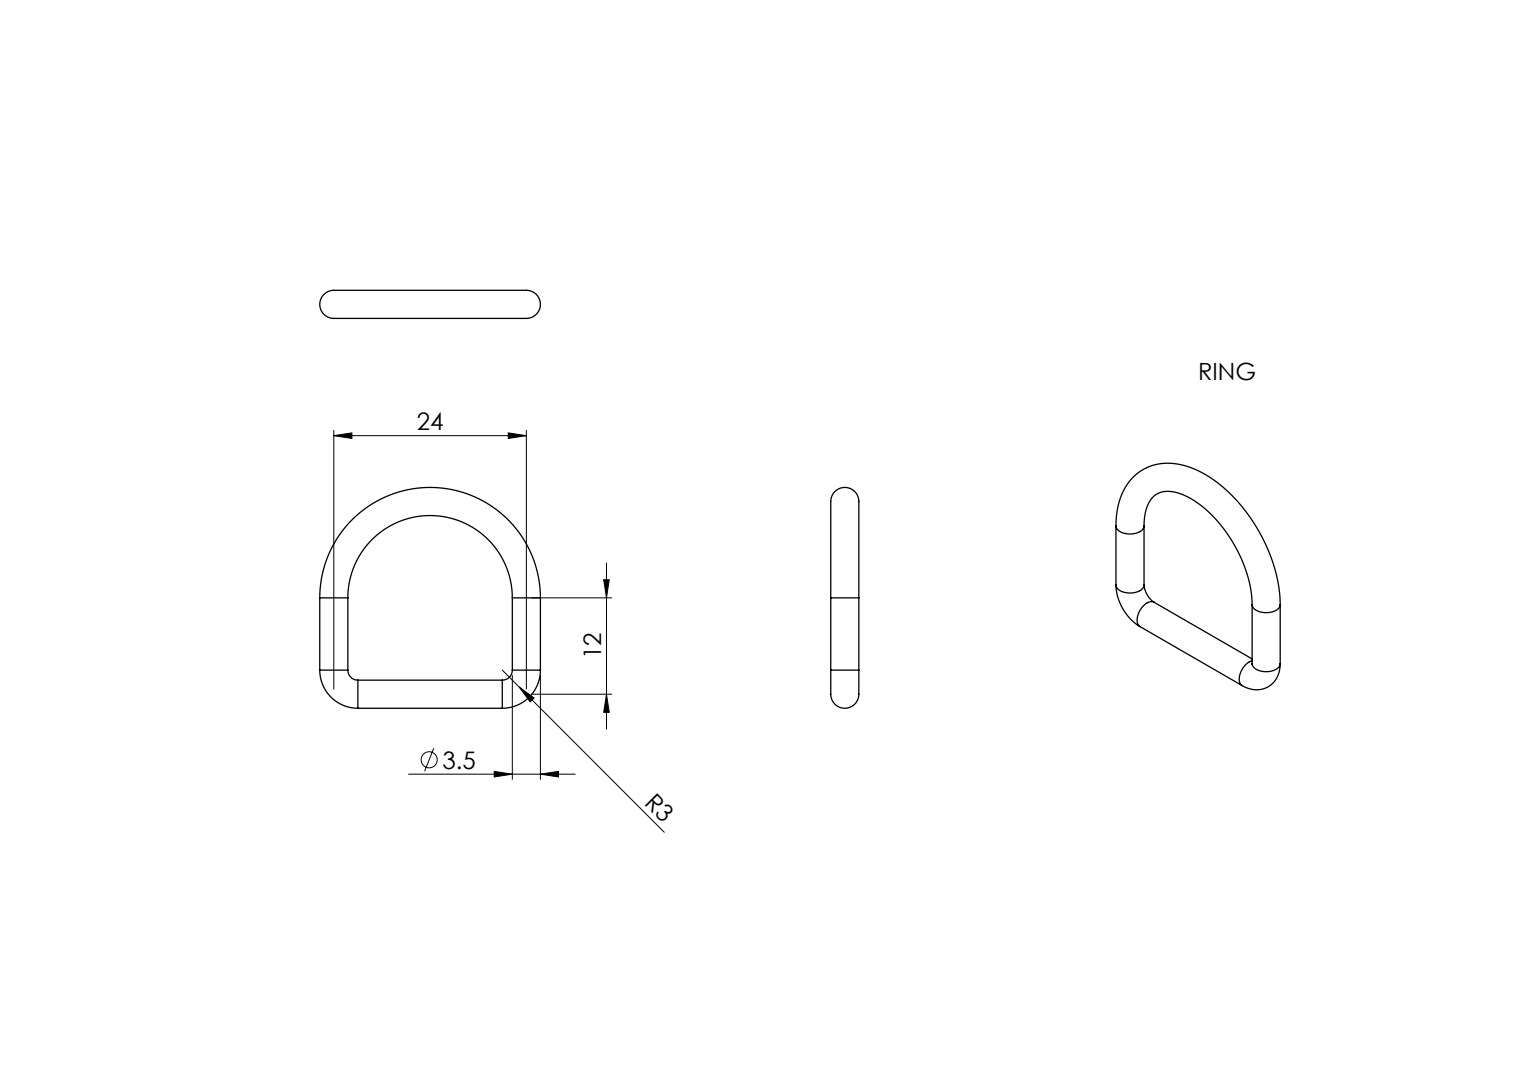
ISO-10303-21;
HEADER;
FILE_DESCRIPTION (('STEP AP214'),
    '1' );
FILE_NAME ('ring.step',
    '2026-10-26T11:20:31',
    ( '' ),
    ( '' ),
    'SwSTEP 2.0',
    'SolidWorks 2026',
    '' );
FILE_SCHEMA (( 'AUTOMOTIVE_DESIGN' ));
ENDSEC;

DATA;
#29=VERTEX_POINT ( 'NONE', #4130 ) ;
#30=CARTESIAN_POINT ( 'NONE',  ( -8.999999999999998224, 36.00000000000000711, 0.000000000000000000 ) ) ;
#48=CIRCLE ( 'NONE', #1190, 1.749999999999999778 ) ;
#49=DIRECTION ( 'NONE',  ( -0.000000000000000000, -0.000000000000000000, -1.000000000000000000 ) ) ;
#66=TOROIDAL_SURFACE ( 'NONE', #1579, 12.00000000000000000, 1.749999999999999778 ) ;
#77=CIRCLE ( 'NONE', #3336, 1.749999999999999778 ) ;
#79=UNCERTAINTY_MEASURE_WITH_UNIT (LENGTH_MEASURE( 1.000000000000000082E-05 ), #706, 'distance_accuracy_value', 'NONE');
#80=DIRECTION ( 'NONE',  ( 1.000000000000000000, -1.621111868633889227E-15, 0.000000000000000000 ) ) ;
#88=FACE_OUTER_BOUND ( 'NONE', #3234, .T. ) ;
#100=CIRCLE ( 'NONE', #1688, 1.749999999999999778 ) ;
#121=( NAMED_UNIT ( * ) PLANE_ANGLE_UNIT ( ) SI_UNIT ( $, .RADIAN. ) );
#148=ORIENTED_EDGE ( 'NONE', *, *, #3909, .T. ) ;
#150=ORIENTED_EDGE ( 'NONE', *, *, #4580, .T. ) ;
#175=CARTESIAN_POINT ( 'NONE',  ( -1.734723475976807094E-15, 45.00000000000000000, 0.000000000000000000 ) ) ;
#218=CIRCLE ( 'NONE', #2726, 1.250000000000002887 ) ;
#228=ORIENTED_EDGE ( 'NONE', *, *, #457, .T. ) ;
#244=CARTESIAN_POINT ( 'NONE',  ( 8.999999999999996447, 34.74999999999999289, 2.143131898507865832E-16 ) ) ;
#261=DIRECTION ( 'NONE',  ( 0.000000000000000000, 0.000000000000000000, 1.000000000000000000 ) ) ;
#303=CARTESIAN_POINT ( 'NONE',  ( 9.000000000000003553, 36.00000000000000000, 2.143131898507868051E-16 ) ) ;
#327=ORIENTED_EDGE ( 'NONE', *, *, #457, .F. ) ;
#344=SHAPE_DEFINITION_REPRESENTATION ( #546, #4641 ) ;
#347=DIRECTION ( 'NONE',  ( -1.000000000000000000, -0.000000000000000000, -0.000000000000000000 ) ) ;
#357=DIRECTION ( 'NONE',  ( -0.000000000000000000, -0.000000000000000000, -1.000000000000000000 ) ) ;
#372=EDGE_LOOP ( 'NONE', ( #1130, #2275, #3372, #4073 ) ) ;
#376=ORIENTED_EDGE ( 'NONE', *, *, #4634, .F. ) ;
#379=LINE ( 'NONE', #4051, #4102 ) ;
#430=DIRECTION ( 'NONE',  ( -1.000000000000000000, 0.000000000000000000, 0.000000000000000000 ) ) ;
#455=CARTESIAN_POINT ( 'NONE',  ( 8.999999999999980460, 32.99999999999999289, 0.000000000000000000 ) ) ;
#457=EDGE_CURVE ( 'NONE', #2385, #2339, #3083, .T. ) ;
#459=EDGE_CURVE ( 'NONE', #2022, #1315, #48, .T. ) ;
#469=EDGE_CURVE ( 'NONE', #29, #4376, #2892, .T. ) ;
#481=UNCERTAINTY_MEASURE_WITH_UNIT (LENGTH_MEASURE( 1.000000000000000082E-05 ), #3442, 'distance_accuracy_value', 'NONE');
#489=CIRCLE ( 'NONE', #2768, 1.750000000000001554 ) ;
#493=CYLINDRICAL_SURFACE ( 'NONE', #995, 1.749999999999999778 ) ;
#522=FILL_AREA_STYLE_COLOUR ( '', #3240 ) ;
#529=( GEOMETRIC_REPRESENTATION_CONTEXT ( 3 ) GLOBAL_UNCERTAINTY_ASSIGNED_CONTEXT ( ( #79 ) ) GLOBAL_UNIT_ASSIGNED_CONTEXT ( ( #706, #2210, #4340 ) ) REPRESENTATION_CONTEXT ( 'NONE', 'WORKASPACE' ) );
#532=CIRCLE ( 'NONE', #3102, 1.750000000000001554 ) ;
#545=CARTESIAN_POINT ( 'NONE',  ( -8.999999999999998224, 36.00000000000000711, 2.143131898507868051E-16 ) ) ;
#546=PRODUCT_DEFINITION_SHAPE ( 'NONE', 'NONE',  #1816 ) ;
#548=EDGE_LOOP ( 'NONE', ( #758, #4521, #1673, #3066 ) ) ;
#579=EDGE_CURVE ( 'NONE', #3730, #2339, #1566, .T. ) ;
#614=VERTEX_POINT ( 'NONE', #1484 ) ;
#615=DIRECTION ( 'NONE',  ( 8.921435019309286191E-15, 1.000000000000000000, 0.000000000000000000 ) ) ;
#619=DIRECTION ( 'NONE',  ( 1.000000000000000000, 0.000000000000000000, 0.000000000000000000 ) ) ;
#636=EDGE_LOOP ( 'NONE', ( #2161, #3608, #3305, #4453 ) ) ;
#655=CARTESIAN_POINT ( 'NONE',  ( 12.00000000000000178, 36.00000000000000000, 0.000000000000000000 ) ) ;
#660=SURFACE_SIDE_STYLE ('',( #3422 ) ) ;
#684=PRODUCT_CONTEXT ( 'NONE', #3739, 'mechanical' ) ;
#690=CARTESIAN_POINT ( 'NONE',  ( 8.999999999999980460, 32.99999999999999289, -1.749999999999999778 ) ) ;
#700=EDGE_LOOP ( 'NONE', ( #4101, #4550, #228, #2693, #3793 ) ) ;
#702=CARTESIAN_POINT ( 'NONE',  ( 9.000000000000003553, 36.00000000000000000, 0.000000000000000000 ) ) ;
#706=( LENGTH_UNIT ( ) NAMED_UNIT ( * ) SI_UNIT ( .MILLI., .METRE. ) );
#713=CARTESIAN_POINT ( 'NONE',  ( 10.25000000000001954, 44.99999999999999289, 2.143131898507868051E-16 ) ) ;
#733=DIRECTION ( 'NONE',  ( 5.782411586589374402E-16, -1.000000000000000000, 0.000000000000000000 ) ) ;
#744=DIRECTION ( 'NONE',  ( -0.000000000000000000, -0.000000000000000000, -1.000000000000000000 ) ) ;
#758=ORIENTED_EDGE ( 'NONE', *, *, #1941, .F. ) ;
#762=DIRECTION ( 'NONE',  ( 1.000000000000000000, -8.560005772541128451E-15, 0.000000000000000000 ) ) ;
#767=CARTESIAN_POINT ( 'NONE',  ( -1.734723475976807094E-15, 45.00000000000000000, 2.143131898507868051E-16 ) ) ;
#768=AXIS2_PLACEMENT_3D ( 'NONE', #3232, #762, #3279 ) ;
#780=CARTESIAN_POINT ( 'NONE',  ( -13.75000000000000178, 36.00000000000001421, 0.000000000000000000 ) ) ;
#787=EDGE_LOOP ( 'NONE', ( #3435, #2481, #1946, #2209, #849 ) ) ;
#836=ORIENTED_EDGE ( 'NONE', *, *, #2413, .T. ) ;
#838=DIRECTION ( 'NONE',  ( 1.000000000000000000, 0.000000000000000000, 0.000000000000000000 ) ) ;
#849=ORIENTED_EDGE ( 'NONE', *, *, #1941, .T. ) ;
#853=AXIS2_PLACEMENT_3D ( 'NONE', #455, #2640, #4104 ) ;
#859=DIRECTION ( 'NONE',  ( -1.428364815747576977E-15, -1.000000000000000000, 0.000000000000000000 ) ) ;
#918=CYLINDRICAL_SURFACE ( 'NONE', #4520, 1.749999999999999778 ) ;
#927=DIRECTION ( 'NONE',  ( 1.621111868633889227E-15, 1.000000000000000000, 0.000000000000000000 ) ) ;
#929=PRESENTATION_STYLE_ASSIGNMENT (( #2652 ) ) ;
#945=DIRECTION ( 'NONE',  ( 1.000000000000000000, 0.000000000000000000, 0.000000000000000000 ) ) ;
#955=AXIS2_PLACEMENT_3D ( 'NONE', #1133, #2645, #3717 ) ;
#958=ORIENTED_EDGE ( 'NONE', *, *, #4634, .T. ) ;
#962=AXIS2_PLACEMENT_3D ( 'NONE', #3454, #3122, #3098 ) ;
#966=CARTESIAN_POINT ( 'NONE',  ( -8.999999999999969802, 34.74999999999999289, 2.143131898507857451E-16 ) ) ;
#971=VECTOR ( 'NONE', #2847, 1000.000000000000000 ) ;
#976=FACE_OUTER_BOUND ( 'NONE', #2756, .T. ) ;
#982=CIRCLE ( 'NONE', #4392, 1.749999999999999778 ) ;
#995=AXIS2_PLACEMENT_3D ( 'NONE', #2650, #4193, #2333 ) ;
#1008=DIRECTION ( 'NONE',  ( 1.000000000000000000, 0.000000000000000000, 0.000000000000000000 ) ) ;
#1032=CARTESIAN_POINT ( 'NONE',  ( 13.75000000000000178, 36.00000000000000000, 0.000000000000000000 ) ) ;
#1057=AXIS2_PLACEMENT_3D ( 'NONE', #767, #357, #430 ) ;
#1058=DIRECTION ( 'NONE',  ( 1.621111868633889227E-15, 1.000000000000000000, 0.000000000000000000 ) ) ;
#1070=EDGE_CURVE ( 'NONE', #4401, #3730, #2816, .T. ) ;
#1083=CLOSED_SHELL ( 'NONE', ( #1845, #4127, #2356, #3065, #4322, #2721, #4192, #3598, #1324, #1603, #2660, #3233 ) ) ;
#1087=DIRECTION ( 'NONE',  ( -1.000000000000000000, 0.000000000000000000, 0.000000000000000000 ) ) ;
#1116=PRODUCT_DEFINITION_FORMATION_WITH_SPECIFIED_SOURCE ( 'ANY', '', #2031, .NOT_KNOWN. ) ;
#1130=ORIENTED_EDGE ( 'NONE', *, *, #4580, .F. ) ;
#1133=CARTESIAN_POINT ( 'NONE',  ( -8.999999999999998224, 36.00000000000000711, 0.000000000000000000 ) ) ;
#1144=( NAMED_UNIT ( * ) PLANE_ANGLE_UNIT ( ) SI_UNIT ( $, .RADIAN. ) );
#1150=TOROIDAL_SURFACE ( 'NONE', #1749, 3.000000000000002665, 1.749999999999999778 ) ;
#1171=CARTESIAN_POINT ( 'NONE',  ( -12.00000000000000178, 36.00000000000001421, 0.000000000000000000 ) ) ;
#1177=EDGE_CURVE ( 'NONE', #3258, #4401, #3344, .T. ) ;
#1178=AXIS2_PLACEMENT_3D ( 'NONE', #175, #3762, #2028 ) ;
#1190=AXIS2_PLACEMENT_3D ( 'NONE', #2109, #1819, #1396 ) ;
#1202=AXIS2_PLACEMENT_3D ( 'NONE', #4076, #80, #3046 ) ;
#1208=AXIS2_PLACEMENT_3D ( 'NONE', #1938, #1277, #945 ) ;
#1237=( NAMED_UNIT ( * ) SI_UNIT ( $, .STERADIAN. ) SOLID_ANGLE_UNIT ( ) );
#1252=CARTESIAN_POINT ( 'NONE',  ( -13.75000000000000178, 44.99999999999999289, 0.000000000000000000 ) ) ;
#1277=DIRECTION ( 'NONE',  ( 5.782411586589374402E-16, -1.000000000000000000, 0.000000000000000000 ) ) ;
#1286=CARTESIAN_POINT ( 'NONE',  ( 12.00000000000000178, 36.00000000000000000, 0.000000000000000000 ) ) ;
#1296=DIRECTION ( 'NONE',  ( -0.000000000000000000, -0.000000000000000000, -1.000000000000000000 ) ) ;
#1298=AXIS2_PLACEMENT_3D ( 'NONE', #3596, #3193, #1008 ) ;
#1313=ORIENTED_EDGE ( 'NONE', *, *, #3981, .T. ) ;
#1315=VERTEX_POINT ( 'NONE', #3475 ) ;
#1324=ADVANCED_FACE ( 'NONE', ( #3097 ), #1150, .T. ) ;
#1347=DIRECTION ( 'NONE',  ( 1.982541115402063335E-15, 1.000000000000000000, 0.000000000000000000 ) ) ;
#1365=FACE_OUTER_BOUND ( 'NONE', #1708, .T. ) ;
#1396=DIRECTION ( 'NONE',  ( -1.000000000000000000, 0.000000000000000000, 0.000000000000000000 ) ) ;
#1401=AXIS2_PLACEMENT_3D ( 'NONE', #655, #1058, #3239 ) ;
#1431=DIRECTION ( 'NONE',  ( 1.000000000000000000, 0.000000000000000000, 0.000000000000000000 ) ) ;
#1472=TOROIDAL_SURFACE ( 'NONE', #955, 3.000000000000002665, 1.749999999999999778 ) ;
#1484=CARTESIAN_POINT ( 'NONE',  ( -8.999999999999973355, 32.99999999999999289, 1.749999999999999778 ) ) ;
#1511=( NAMED_UNIT ( * ) SI_UNIT ( $, .STERADIAN. ) SOLID_ANGLE_UNIT ( ) );
#1536=ORIENTED_EDGE ( 'NONE', *, *, #3804, .T. ) ;
#1554=AXIS2_PLACEMENT_3D ( 'NONE', #3843, #2742, #3798 ) ;
#1566=CIRCLE ( 'NONE', #3162, 1.750000000000001554 ) ;
#1579=AXIS2_PLACEMENT_3D ( 'NONE', #1616, #2659, #4176 ) ;
#1603=ADVANCED_FACE ( 'NONE', ( #3825 ), #493, .T. ) ;
#1609=AXIS2_PLACEMENT_3D ( 'NONE', #702, #744, #2587 ) ;
#1616=CARTESIAN_POINT ( 'NONE',  ( -1.734723475976807094E-15, 45.00000000000000000, 0.000000000000000000 ) ) ;
#1628=LINE ( 'NONE', #4189, #3221 ) ;
#1632=SHAPE_REPRESENTATION_RELATIONSHIP ( 'NONE' , 'NONE' ,  #4641, #4382 ) ;
#1643=VERTEX_POINT ( 'NONE', #3398 ) ;
#1663=DIRECTION ( 'NONE',  ( -1.000000000000000000, -0.000000000000000000, -0.000000000000000000 ) ) ;
#1664=CARTESIAN_POINT ( 'NONE',  ( -8.999999999999998224, 36.00000000000000711, 0.000000000000000000 ) ) ;
#1673=ORIENTED_EDGE ( 'NONE', *, *, #3531, .T. ) ;
#1685=ORIENTED_EDGE ( 'NONE', *, *, #3593, .T. ) ;
#1688=AXIS2_PLACEMENT_3D ( 'NONE', #4667, #1726, #4615 ) ;
#1703=EDGE_CURVE ( 'NONE', #1315, #2022, #100, .T. ) ;
#1708=EDGE_LOOP ( 'NONE', ( #3770, #2507, #1313, #2365 ) ) ;
#1712=DIRECTION ( 'NONE',  ( 0.000000000000000000, 0.000000000000000000, 1.000000000000000000 ) ) ;
#1717=CARTESIAN_POINT ( 'NONE',  ( 8.999999999999966249, 31.24999999999999645, 0.000000000000000000 ) ) ;
#1726=DIRECTION ( 'NONE',  ( 1.621111868633889227E-15, 1.000000000000000000, 0.000000000000000000 ) ) ;
#1727=DIRECTION ( 'NONE',  ( -1.428364815747576977E-15, -1.000000000000000000, 0.000000000000000000 ) ) ;
#1749=AXIS2_PLACEMENT_3D ( 'NONE', #1664, #1296, #3121 ) ;
#1752=LINE ( 'NONE', #713, #3072 ) ;
#1766=CARTESIAN_POINT ( 'NONE',  ( -10.25000000000000178, 44.99999999999999289, 2.143131898507868051E-16 ) ) ;
#1772=FACE_OUTER_BOUND ( 'NONE', #4019, .T. ) ;
#1780=CARTESIAN_POINT ( 'NONE',  ( 0.000000000000000000, 0.000000000000000000, 0.000000000000000000 ) ) ;
#1797=CARTESIAN_POINT ( 'NONE',  ( -10.25000000000000000, 36.00000000000001421, 2.143131898507868051E-16 ) ) ;
#1808=DIRECTION ( 'NONE',  ( -1.000000000000000000, -0.000000000000000000, -0.000000000000000000 ) ) ;
#1816=PRODUCT_DEFINITION ( 'UNKNOWN', '', #1116, #3380 ) ;
#1819=DIRECTION ( 'NONE',  ( 1.621111868633889227E-15, 1.000000000000000000, 0.000000000000000000 ) ) ;
#1840=DIRECTION ( 'NONE',  ( -0.000000000000000000, -0.000000000000000000, -1.000000000000000000 ) ) ;
#1845=ADVANCED_FACE ( 'NONE', ( #976 ), #3736, .T. ) ;
#1861=CARTESIAN_POINT ( 'NONE',  ( 8.999999999999980460, 32.99999999999999289, 1.749999999999999778 ) ) ;
#1875=ORIENTED_EDGE ( 'NONE', *, *, #459, .T. ) ;
#1885=ORIENTED_EDGE ( 'NONE', *, *, #4427, .T. ) ;
#1889=STYLED_ITEM('',(#4729),#2976);
#1894=DIRECTION ( 'NONE',  ( 8.921435019309286191E-15, 1.000000000000000000, 0.000000000000000000 ) ) ;
#1938=CARTESIAN_POINT ( 'NONE',  ( 12.00000000000001954, 44.99999999999999289, 0.000000000000000000 ) ) ;
#1940=TOROIDAL_SURFACE ( 'NONE', #1554, 2.999999999999999112, 1.749999999999999778 ) ;
#1941=EDGE_CURVE ( 'NONE', #29, #3785, #4129, .T. ) ;
#1944=DIRECTION ( 'NONE',  ( 1.982541115402063335E-15, 1.000000000000000000, 0.000000000000000000 ) ) ;
#1946=ORIENTED_EDGE ( 'NONE', *, *, #2540, .F. ) ;
#1960=UNCERTAINTY_MEASURE_WITH_UNIT (LENGTH_MEASURE( 1.000000000000000082E-05 ), #3300, 'distance_accuracy_value', 'NONE');
#1966=CARTESIAN_POINT ( 'NONE',  ( -12.00000000000000000, 36.00000000000001421, 0.000000000000000000 ) ) ;
#1982=ORIENTED_EDGE ( 'NONE', *, *, #2540, .T. ) ;
#1999=EDGE_CURVE ( 'NONE', #4090, #4401, #2905, .T. ) ;
#2020=EDGE_LOOP ( 'NONE', ( #3493, #4114, #148, #4203 ) ) ;
#2022=VERTEX_POINT ( 'NONE', #3024 ) ;
#2028=DIRECTION ( 'NONE',  ( -1.000000000000000000, 0.000000000000000000, 0.000000000000000000 ) ) ;
#2031=PRODUCT ( 'ring', 'ring', '', ( #684 ) ) ;
#2044=VERTEX_POINT ( 'NONE', #1252 ) ;
#2052=CARTESIAN_POINT ( 'NONE',  ( -8.999999999999973355, 32.99999999999999289, 0.000000000000000000 ) ) ;
#2097=AXIS2_PLACEMENT_3D ( 'NONE', #303, #4669, #3948 ) ;
#2109=CARTESIAN_POINT ( 'NONE',  ( 11.99999999999999822, 45.00000000000000000, 0.000000000000000000 ) ) ;
#2161=ORIENTED_EDGE ( 'NONE', *, *, #1703, .F. ) ;
#2175=LINE ( 'NONE', #2504, #3837 ) ;
#2196=VERTEX_POINT ( 'NONE', #966 ) ;
#2209=ORIENTED_EDGE ( 'NONE', *, *, #3457, .T. ) ;
#2210=( NAMED_UNIT ( * ) PLANE_ANGLE_UNIT ( ) SI_UNIT ( $, .RADIAN. ) );
#2224=ORIENTED_EDGE ( 'NONE', *, *, #2866, .F. ) ;
#2241=CARTESIAN_POINT ( 'NONE',  ( -8.999999999999973355, 32.99999999999999289, -1.749999999999999778 ) ) ;
#2242=CARTESIAN_POINT ( 'NONE',  ( 8.999999999999980460, 32.99999999999999289, 0.000000000000000000 ) ) ;
#2258=ORIENTED_EDGE ( 'NONE', *, *, #2392, .T. ) ;
#2274=ORIENTED_EDGE ( 'NONE', *, *, #2392, .F. ) ;
#2275=ORIENTED_EDGE ( 'NONE', *, *, #3531, .F. ) ;
#2320=FACE_OUTER_BOUND ( 'NONE', #372, .T. ) ;
#2333=DIRECTION ( 'NONE',  ( -1.000000000000000000, 0.000000000000000000, 0.000000000000000000 ) ) ;
#2337=ORIENTED_EDGE ( 'NONE', *, *, #579, .T. ) ;
#2339=VERTEX_POINT ( 'NONE', #244 ) ;
#2356=ADVANCED_FACE ( 'NONE', ( #2418 ), #3661, .T. ) ;
#2365=ORIENTED_EDGE ( 'NONE', *, *, #3432, .T. ) ;
#2385=VERTEX_POINT ( 'NONE', #3640 ) ;
#2392=EDGE_CURVE ( 'NONE', #4090, #614, #379, .T. ) ;
#2413=EDGE_CURVE ( 'NONE', #1643, #3785, #4471, .T. ) ;
#2418=FACE_OUTER_BOUND ( 'NONE', #2917, .T. ) ;
#2435=FACE_OUTER_BOUND ( 'NONE', #4002, .T. ) ;
#2449=EDGE_CURVE ( 'NONE', #4376, #1315, #3552, .T. ) ;
#2454=CARTESIAN_POINT ( 'NONE',  ( 8.999999999999984013, 32.99999999999999289, 0.000000000000000000 ) ) ;
#2463=ORIENTED_EDGE ( 'NONE', *, *, #2449, .F. ) ;
#2468=DIRECTION ( 'NONE',  ( -1.621111868633889227E-15, -1.000000000000000000, 0.000000000000000000 ) ) ;
#2481=ORIENTED_EDGE ( 'NONE', *, *, #3804, .F. ) ;
#2492=CIRCLE ( 'NONE', #3715, 1.749999999999999778 ) ;
#2493=DIRECTION ( 'NONE',  ( 1.000000000000000000, -1.621111868633889227E-15, 0.000000000000000000 ) ) ;
#2504=CARTESIAN_POINT ( 'NONE',  ( 8.999999999999984013, 32.99999999999999289, -1.749999999999999778 ) ) ;
#2507=ORIENTED_EDGE ( 'NONE', *, *, #459, .F. ) ;
#2540=EDGE_CURVE ( 'NONE', #2196, #614, #3249, .T. ) ;
#2561=DIRECTION ( 'NONE',  ( -0.000000000000000000, -0.000000000000000000, -1.000000000000000000 ) ) ;
#2578=AXIS2_PLACEMENT_3D ( 'NONE', #3727, #49, #2948 ) ;
#2587=DIRECTION ( 'NONE',  ( -1.000000000000000000, 0.000000000000000000, 0.000000000000000000 ) ) ;
#2599=EDGE_CURVE ( 'NONE', #2044, #4376, #982, .T. ) ;
#2640=DIRECTION ( 'NONE',  ( 1.000000000000000000, -8.560005772541128451E-15, 0.000000000000000000 ) ) ;
#2645=DIRECTION ( 'NONE',  ( -0.000000000000000000, -0.000000000000000000, -1.000000000000000000 ) ) ;
#2650=CARTESIAN_POINT ( 'NONE',  ( -12.00000000000000000, 36.00000000000001421, 0.000000000000000000 ) ) ;
#2652=SURFACE_STYLE_USAGE ( .BOTH. , #660 ) ;
#2659=DIRECTION ( 'NONE',  ( -0.000000000000000000, -0.000000000000000000, -1.000000000000000000 ) ) ;
#2660=ADVANCED_FACE ( 'NONE', ( #2320 ), #66, .T. ) ;
#2693=ORIENTED_EDGE ( 'NONE', *, *, #2866, .T. ) ;
#2721=ADVANCED_FACE ( 'NONE', ( #2435 ), #3516, .T. ) ;
#2726=AXIS2_PLACEMENT_3D ( 'NONE', #545, #4168, #3135 ) ;
#2742=DIRECTION ( 'NONE',  ( -0.000000000000000000, -0.000000000000000000, -1.000000000000000000 ) ) ;
#2756=EDGE_LOOP ( 'NONE', ( #3809, #150, #1875, #2463 ) ) ;
#2768=AXIS2_PLACEMENT_3D ( 'NONE', #3366, #3695, #1944 ) ;
#2777=ORIENTED_EDGE ( 'NONE', *, *, #1070, .T. ) ;
#2816=CIRCLE ( 'NONE', #768, 1.750000000000001554 ) ;
#2818=CARTESIAN_POINT ( 'NONE',  ( 13.75000000000001954, 44.99999999999999289, 0.000000000000000000 ) ) ;
#2819=FILL_AREA_STYLE ('',( #522 ) ) ;
#2826=ORIENTED_EDGE ( 'NONE', *, *, #1177, .T. ) ;
#2847=DIRECTION ( 'NONE',  ( -1.927470528863123239E-16, 1.000000000000000000, 0.000000000000000000 ) ) ;
#2858=DIRECTION ( 'NONE',  ( -1.000000000000000000, 0.000000000000000000, 0.000000000000000000 ) ) ;
#2866=EDGE_CURVE ( 'NONE', #2339, #4090, #4250, .T. ) ;
#2892=LINE ( 'NONE', #1797, #971 ) ;
#2905=CIRCLE ( 'NONE', #853, 1.750000000000001554 ) ;
#2917=EDGE_LOOP ( 'NONE', ( #4444, #2826, #2777, #2337, #327 ) ) ;
#2928=AXIS2_PLACEMENT_3D ( 'NONE', #1780, #1712, #3957 ) ;
#2948=DIRECTION ( 'NONE',  ( -1.000000000000000000, 0.000000000000000000, 0.000000000000000000 ) ) ;
#2976=MANIFOLD_SOLID_BREP ( 'Sweep1', #1083 ) ;
#2979=ORIENTED_EDGE ( 'NONE', *, *, #1999, .F. ) ;
#2997=ORIENTED_EDGE ( 'NONE', *, *, #3593, .F. ) ;
#3024=CARTESIAN_POINT ( 'NONE',  ( 13.74999999999999822, 45.00000000000000000, 0.000000000000000000 ) ) ;
#3046=DIRECTION ( 'NONE',  ( 1.982541115402063335E-15, 1.000000000000000000, 0.000000000000000000 ) ) ;
#3065=ADVANCED_FACE ( 'NONE', ( #4486 ), #4206, .T. ) ;
#3066=ORIENTED_EDGE ( 'NONE', *, *, #3909, .F. ) ;
#3072=VECTOR ( 'NONE', #733, 1000.000000000000000 ) ;
#3081=DIRECTION ( 'NONE',  ( -1.927470528863123239E-16, 1.000000000000000000, 0.000000000000000000 ) ) ;
#3083=CIRCLE ( 'NONE', #2097, 1.249999999999999334 ) ;
#3097=FACE_OUTER_BOUND ( 'NONE', #787, .T. ) ;
#3098=DIRECTION ( 'NONE',  ( 1.982541115402063335E-15, 1.000000000000000000, 0.000000000000000000 ) ) ;
#3102=AXIS2_PLACEMENT_3D ( 'NONE', #2052, #2493, #1347 ) ;
#3121=DIRECTION ( 'NONE',  ( -1.000000000000000000, 0.000000000000000000, 0.000000000000000000 ) ) ;
#3122=DIRECTION ( 'NONE',  ( 1.000000000000000000, -1.621111868633889227E-15, 0.000000000000000000 ) ) ;
#3135=DIRECTION ( 'NONE',  ( -1.000000000000000000, 0.000000000000000000, 0.000000000000000000 ) ) ;
#3162=AXIS2_PLACEMENT_3D ( 'NONE', #2242, #3696, #1894 ) ;
#3176=AXIS2_PLACEMENT_3D ( 'NONE', #4546, #1663, #261 ) ;
#3193=DIRECTION ( 'NONE',  ( 5.782411586589374402E-16, -1.000000000000000000, 0.000000000000000000 ) ) ;
#3221=VECTOR ( 'NONE', #3081, 1000.000000000000000 ) ;
#3226=CIRCLE ( 'NONE', #1178, 13.75000000000000000 ) ;
#3232=CARTESIAN_POINT ( 'NONE',  ( 8.999999999999980460, 32.99999999999999289, 0.000000000000000000 ) ) ;
#3233=ADVANCED_FACE ( 'NONE', ( #1365 ), #3906, .T. ) ;
#3234=EDGE_LOOP ( 'NONE', ( #3755, #836, #1885, #3613, #376 ) ) ;
#3239=DIRECTION ( 'NONE',  ( -1.000000000000000000, 0.000000000000000000, 0.000000000000000000 ) ) ;
#3240=COLOUR_RGB ( '',0.8941176470588234615, 0.8941176470588234615, 0.8941176470588234615 ) ;
#3246=EDGE_CURVE ( 'NONE', #1643, #3829, #532, .T. ) ;
#3249=CIRCLE ( 'NONE', #1202, 1.750000000000001554 ) ;
#3258=VERTEX_POINT ( 'NONE', #1032 ) ;
#3263=CARTESIAN_POINT ( 'NONE',  ( -12.00000000000000178, 36.00000000000001421, 0.000000000000000000 ) ) ;
#3279=DIRECTION ( 'NONE',  ( 8.921435019309286191E-15, 1.000000000000000000, 0.000000000000000000 ) ) ;
#3300=( LENGTH_UNIT ( ) NAMED_UNIT ( * ) SI_UNIT ( .MILLI., .METRE. ) );
#3305=ORIENTED_EDGE ( 'NONE', *, *, #4413, .T. ) ;
#3336=AXIS2_PLACEMENT_3D ( 'NONE', #1286, #927, #3441 ) ;
#3344=CIRCLE ( 'NONE', #2578, 4.749999999999999112 ) ;
#3366=CARTESIAN_POINT ( 'NONE',  ( -8.999999999999973355, 32.99999999999999289, 0.000000000000000000 ) ) ;
#3372=ORIENTED_EDGE ( 'NONE', *, *, #2449, .T. ) ;
#3380=PRODUCT_DEFINITION_CONTEXT ( 'detailed design', #3583, 'design' ) ;
#3391=MECHANICAL_DESIGN_GEOMETRIC_PRESENTATION_REPRESENTATION('',(#4696),#4310);
#3398=CARTESIAN_POINT ( 'NONE',  ( -8.999999999999976907, 31.24999999999999645, 0.000000000000000000 ) ) ;
#3422=SURFACE_STYLE_FILL_AREA ( #2819 ) ;
#3428=CARTESIAN_POINT ( 'NONE',  ( -12.00000000000000178, 44.99999999999999289, 0.000000000000000000 ) ) ;
#3432=EDGE_CURVE ( 'NONE', #3258, #2385, #77, .T. ) ;
#3435=ORIENTED_EDGE ( 'NONE', *, *, #2413, .F. ) ;
#3441=DIRECTION ( 'NONE',  ( -1.000000000000000000, 0.000000000000000000, 0.000000000000000000 ) ) ;
#3442=( LENGTH_UNIT ( ) NAMED_UNIT ( * ) SI_UNIT ( .MILLI., .METRE. ) );
#3454=CARTESIAN_POINT ( 'NONE',  ( -8.999999999999973355, 32.99999999999999289, 0.000000000000000000 ) ) ;
#3456=CIRCLE ( 'NONE', #1401, 1.749999999999999778 ) ;
#3457=EDGE_CURVE ( 'NONE', #2196, #29, #218, .T. ) ;
#3460=FACE_OUTER_BOUND ( 'NONE', #548, .T. ) ;
#3475=CARTESIAN_POINT ( 'NONE',  ( 10.24999999999999822, 45.00000000000000000, 2.143131898507898126E-16 ) ) ;
#3493=ORIENTED_EDGE ( 'NONE', *, *, #469, .F. ) ;
#3504=CARTESIAN_POINT ( 'NONE',  ( 8.999999999999980460, 32.99999999999999289, 0.000000000000000000 ) ) ;
#3516=CYLINDRICAL_SURFACE ( 'NONE', #3176, 1.749999999999999778 ) ;
#3531=EDGE_CURVE ( 'NONE', #4376, #2044, #2492, .T. ) ;
#3552=CIRCLE ( 'NONE', #1057, 10.25000000000000000 ) ;
#3583=APPLICATION_CONTEXT ( 'automotive_design' ) ;
#3593=EDGE_CURVE ( 'NONE', #3730, #3829, #2175, .T. ) ;
#3596=CARTESIAN_POINT ( 'NONE',  ( 12.00000000000001954, 44.99999999999999289, 0.000000000000000000 ) ) ;
#3598=ADVANCED_FACE ( 'NONE', ( #1772 ), #3970, .T. ) ;
#3600=LINE ( 'NONE', #2818, #4068 ) ;
#3605=DIRECTION ( 'NONE',  ( 0.000000000000000000, 0.000000000000000000, 1.000000000000000000 ) ) ;
#3607=CIRCLE ( 'NONE', #962, 1.750000000000001554 ) ;
#3608=ORIENTED_EDGE ( 'NONE', *, *, #3705, .T. ) ;
#3613=ORIENTED_EDGE ( 'NONE', *, *, #3457, .F. ) ;
#3640=CARTESIAN_POINT ( 'NONE',  ( 10.25000000000000178, 36.00000000000000000, 2.143131898507893689E-16 ) ) ;
#3655=AXIS2_PLACEMENT_3D ( 'NONE', #3990, #1840, #1087 ) ;
#3661=TOROIDAL_SURFACE ( 'NONE', #1609, 2.999999999999999112, 1.749999999999999778 ) ;
#3695=DIRECTION ( 'NONE',  ( 1.000000000000000000, -1.621111868633889227E-15, 0.000000000000000000 ) ) ;
#3696=DIRECTION ( 'NONE',  ( 1.000000000000000000, -8.560005772541128451E-15, 0.000000000000000000 ) ) ;
#3705=EDGE_CURVE ( 'NONE', #1315, #2385, #1752, .T. ) ;
#3712=DIRECTION ( 'NONE',  ( 1.000000000000000000, 0.000000000000000000, 0.000000000000000000 ) ) ;
#3713=MECHANICAL_DESIGN_GEOMETRIC_PRESENTATION_REPRESENTATION('',(#1889),#529);
#3715=AXIS2_PLACEMENT_3D ( 'NONE', #3895, #1727, #619 ) ;
#3717=DIRECTION ( 'NONE',  ( -1.000000000000000000, 0.000000000000000000, 0.000000000000000000 ) ) ;
#3727=CARTESIAN_POINT ( 'NONE',  ( 9.000000000000003553, 36.00000000000000000, 0.000000000000000000 ) ) ;
#3730=VERTEX_POINT ( 'NONE', #690 ) ;
#3736=TOROIDAL_SURFACE ( 'NONE', #3655, 12.00000000000000000, 1.749999999999999778 ) ;
#3739=APPLICATION_CONTEXT ( 'automotive_design' ) ;
#3755=ORIENTED_EDGE ( 'NONE', *, *, #3246, .F. ) ;
#3762=DIRECTION ( 'NONE',  ( -0.000000000000000000, -0.000000000000000000, -1.000000000000000000 ) ) ;
#3770=ORIENTED_EDGE ( 'NONE', *, *, #3705, .F. ) ;
#3775=( GEOMETRIC_REPRESENTATION_CONTEXT ( 3 ) GLOBAL_UNCERTAINTY_ASSIGNED_CONTEXT ( ( #1960 ) ) GLOBAL_UNIT_ASSIGNED_CONTEXT ( ( #3300, #1144, #1511 ) ) REPRESENTATION_CONTEXT ( 'NONE', 'WORKASPACE' ) );
#3785=VERTEX_POINT ( 'NONE', #780 ) ;
#3793=ORIENTED_EDGE ( 'NONE', *, *, #1999, .T. ) ;
#3798=DIRECTION ( 'NONE',  ( -1.000000000000000000, 0.000000000000000000, 0.000000000000000000 ) ) ;
#3804=EDGE_CURVE ( 'NONE', #614, #1643, #489, .T. ) ;
#3809=ORIENTED_EDGE ( 'NONE', *, *, #2599, .F. ) ;
#3825=FACE_OUTER_BOUND ( 'NONE', #2020, .T. ) ;
#3829=VERTEX_POINT ( 'NONE', #2241 ) ;
#3837=VECTOR ( 'NONE', #347, 1000.000000000000000 ) ;
#3843=CARTESIAN_POINT ( 'NONE',  ( 9.000000000000003553, 36.00000000000000000, 0.000000000000000000 ) ) ;
#3869=AXIS2_PLACEMENT_3D ( 'NONE', #3504, #4633, #615 ) ;
#3895=CARTESIAN_POINT ( 'NONE',  ( -12.00000000000000178, 44.99999999999999289, 0.000000000000000000 ) ) ;
#3906=CYLINDRICAL_SURFACE ( 'NONE', #1298, 1.749999999999999778 ) ;
#3909=EDGE_CURVE ( 'NONE', #3785, #2044, #1628, .T. ) ;
#3948=DIRECTION ( 'NONE',  ( -1.000000000000000000, 0.000000000000000000, 0.000000000000000000 ) ) ;
#3957=DIRECTION ( 'NONE',  ( 1.000000000000000000, 0.000000000000000000, 0.000000000000000000 ) ) ;
#3970=CYLINDRICAL_SURFACE ( 'NONE', #4062, 1.749999999999999778 ) ;
#3981=EDGE_CURVE ( 'NONE', #2022, #3258, #3600, .T. ) ;
#3989=CIRCLE ( 'NONE', #4602, 1.749999999999999778 ) ;
#3990=CARTESIAN_POINT ( 'NONE',  ( -1.734723475976807094E-15, 45.00000000000000000, 0.000000000000000000 ) ) ;
#4002=EDGE_LOOP ( 'NONE', ( #4172, #1685, #958, #1982, #2274, #2224 ) ) ;
#4019=EDGE_LOOP ( 'NONE', ( #2997, #4541, #2979, #2258, #1536, #4544 ) ) ;
#4051=CARTESIAN_POINT ( 'NONE',  ( 8.999999999999984013, 32.99999999999999289, 1.749999999999999778 ) ) ;
#4052=DIRECTION ( 'NONE',  ( -1.621111868633889227E-15, -1.000000000000000000, 0.000000000000000000 ) ) ;
#4062=AXIS2_PLACEMENT_3D ( 'NONE', #2454, #4281, #3605 ) ;
#4068=VECTOR ( 'NONE', #4276, 1000.000000000000000 ) ;
#4073=ORIENTED_EDGE ( 'NONE', *, *, #1703, .T. ) ;
#4076=CARTESIAN_POINT ( 'NONE',  ( -8.999999999999973355, 32.99999999999999289, 0.000000000000000000 ) ) ;
#4090=VERTEX_POINT ( 'NONE', #1861 ) ;
#4101=ORIENTED_EDGE ( 'NONE', *, *, #1177, .F. ) ;
#4102=VECTOR ( 'NONE', #1808, 1000.000000000000000 ) ;
#4104=DIRECTION ( 'NONE',  ( 8.921435019309286191E-15, 1.000000000000000000, 0.000000000000000000 ) ) ;
#4114=ORIENTED_EDGE ( 'NONE', *, *, #4427, .F. ) ;
#4127=ADVANCED_FACE ( 'NONE', ( #88 ), #1472, .T. ) ;
#4129=CIRCLE ( 'NONE', #4275, 1.749999999999999778 ) ;
#4130=CARTESIAN_POINT ( 'NONE',  ( -10.25000000000000178, 36.00000000000001421, 2.143131898507868051E-16 ) ) ;
#4157=DIRECTION ( 'NONE',  ( -1.000000000000000000, 0.000000000000000000, 0.000000000000000000 ) ) ;
#4168=DIRECTION ( 'NONE',  ( -0.000000000000000000, -0.000000000000000000, -1.000000000000000000 ) ) ;
#4172=ORIENTED_EDGE ( 'NONE', *, *, #579, .F. ) ;
#4176=DIRECTION ( 'NONE',  ( -1.000000000000000000, 0.000000000000000000, 0.000000000000000000 ) ) ;
#4181=AXIS2_PLACEMENT_3D ( 'NONE', #30, #2561, #2858 ) ;
#4189=CARTESIAN_POINT ( 'NONE',  ( -13.75000000000000000, 36.00000000000001421, 0.000000000000000000 ) ) ;
#4192=ADVANCED_FACE ( 'NONE', ( #4558 ), #1940, .T. ) ;
#4193=DIRECTION ( 'NONE',  ( -1.927470528863123239E-16, 1.000000000000000000, 0.000000000000000000 ) ) ;
#4203=ORIENTED_EDGE ( 'NONE', *, *, #2599, .T. ) ;
#4206=CYLINDRICAL_SURFACE ( 'NONE', #1208, 1.749999999999999778 ) ;
#4250=CIRCLE ( 'NONE', #3869, 1.750000000000001554 ) ;
#4275=AXIS2_PLACEMENT_3D ( 'NONE', #1171, #4052, #3712 ) ;
#4276=DIRECTION ( 'NONE',  ( 5.782411586589374402E-16, -1.000000000000000000, 0.000000000000000000 ) ) ;
#4281=DIRECTION ( 'NONE',  ( -1.000000000000000000, -0.000000000000000000, -0.000000000000000000 ) ) ;
#4310=( GEOMETRIC_REPRESENTATION_CONTEXT ( 3 ) GLOBAL_UNCERTAINTY_ASSIGNED_CONTEXT ( ( #481 ) ) GLOBAL_UNIT_ASSIGNED_CONTEXT ( ( #3442, #121, #1237 ) ) REPRESENTATION_CONTEXT ( 'NONE', 'WORKASPACE' ) );
#4322=ADVANCED_FACE ( 'NONE', ( #3460 ), #918, .T. ) ;
#4340=( NAMED_UNIT ( * ) SI_UNIT ( $, .STERADIAN. ) SOLID_ANGLE_UNIT ( ) );
#4376=VERTEX_POINT ( 'NONE', #1766 ) ;
#4382=ADVANCED_BREP_SHAPE_REPRESENTATION ( '', ( #2976, #2928 ), #3775 ) ;
#4392=AXIS2_PLACEMENT_3D ( 'NONE', #3428, #859, #838 ) ;
#4401=VERTEX_POINT ( 'NONE', #1717 ) ;
#4413=EDGE_CURVE ( 'NONE', #2385, #3258, #3456, .T. ) ;
#4427=EDGE_CURVE ( 'NONE', #3785, #29, #3989, .T. ) ;
#4444=ORIENTED_EDGE ( 'NONE', *, *, #3432, .F. ) ;
#4453=ORIENTED_EDGE ( 'NONE', *, *, #3981, .F. ) ;
#4471=CIRCLE ( 'NONE', #4181, 4.750000000000002665 ) ;
#4486=FACE_OUTER_BOUND ( 'NONE', #636, .T. ) ;
#4520=AXIS2_PLACEMENT_3D ( 'NONE', #1966, #4605, #4157 ) ;
#4521=ORIENTED_EDGE ( 'NONE', *, *, #469, .T. ) ;
#4541=ORIENTED_EDGE ( 'NONE', *, *, #1070, .F. ) ;
#4544=ORIENTED_EDGE ( 'NONE', *, *, #3246, .T. ) ;
#4546=CARTESIAN_POINT ( 'NONE',  ( 8.999999999999984013, 32.99999999999999289, 0.000000000000000000 ) ) ;
#4550=ORIENTED_EDGE ( 'NONE', *, *, #4413, .F. ) ;
#4558=FACE_OUTER_BOUND ( 'NONE', #700, .T. ) ;
#4580=EDGE_CURVE ( 'NONE', #2044, #2022, #3226, .T. ) ;
#4602=AXIS2_PLACEMENT_3D ( 'NONE', #3263, #2468, #1431 ) ;
#4605=DIRECTION ( 'NONE',  ( -1.927470528863123239E-16, 1.000000000000000000, 0.000000000000000000 ) ) ;
#4615=DIRECTION ( 'NONE',  ( -1.000000000000000000, 0.000000000000000000, 0.000000000000000000 ) ) ;
#4633=DIRECTION ( 'NONE',  ( 1.000000000000000000, -8.560005772541128451E-15, 0.000000000000000000 ) ) ;
#4634=EDGE_CURVE ( 'NONE', #3829, #2196, #3607, .T. ) ;
#4641=SHAPE_REPRESENTATION ( 'ring', ( #2928 ), #3775 ) ;
#4667=CARTESIAN_POINT ( 'NONE',  ( 11.99999999999999822, 45.00000000000000000, 0.000000000000000000 ) ) ;
#4669=DIRECTION ( 'NONE',  ( -0.000000000000000000, -0.000000000000000000, -1.000000000000000000 ) ) ;
#4696=STYLED_ITEM ( 'NONE', ( #929 ), #4382 ) ;
#4723=COLOUR_RGB('Light Blue',0.38,0.62,0.78);
#4724=FILL_AREA_STYLE_COLOUR('',#4723);
#4725=FILL_AREA_STYLE('',(#4724));
#4726=SURFACE_STYLE_FILL_AREA(#4725);
#4727=SURFACE_SIDE_STYLE('',(#4726));
#4728=SURFACE_STYLE_USAGE(.BOTH.,#4727);
#4729=PRESENTATION_STYLE_ASSIGNMENT((#4728));
ENDSEC;
END-ISO-10303-21;
